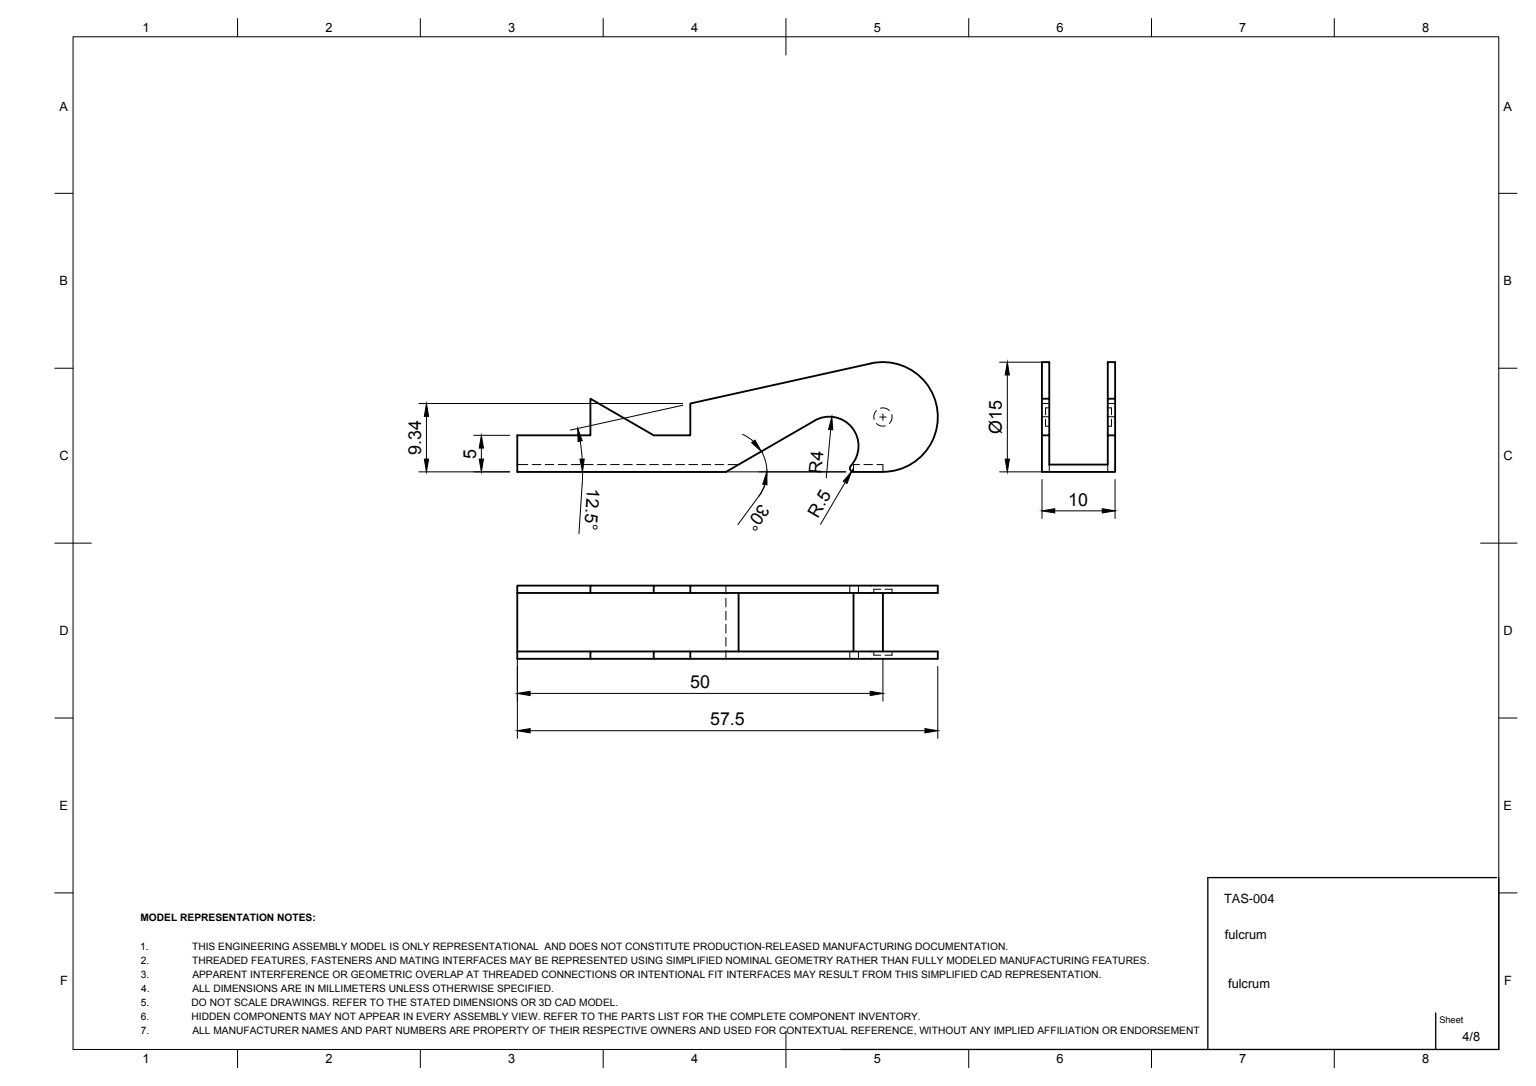
ISO-10303-21;
HEADER;
/* Generated by software containing ST-Developer
 * from STEP Tools, Inc. (www.steptools.com) 
 */

FILE_DESCRIPTION(
/* description */ ('STEP AP214'),
/* implementation_level */ '2;1');

FILE_NAME(
/* name */ 'fulcrum.step',
/* time_stamp */ '2026-11-04T19:48:07-08:00',
/* author */ (''),
/* organization */ (''),
/* preprocessor_version */ 'ST-DEVELOPER v20.2',
/* originating_system */ 'Autodesk Translation Framework v15.17.0.0',
/* authorisation */ '');

FILE_SCHEMA (('AUTOMOTIVE_DESIGN { 1 0 10303 214 3 1 1 }'));
ENDSEC;

DATA;
#10=MECHANICAL_DESIGN_GEOMETRIC_PRESENTATION_REPRESENTATION('',(#60),#9561);
#48=SHAPE_REPRESENTATION_RELATIONSHIP('SRR','None',#9588,#54);
#54=ADVANCED_BREP_SHAPE_REPRESENTATION('',(#66),#9556);
#60=STYLED_ITEM('',(#9627),#66);
#66=MANIFOLD_SOLID_BREP('Body1',#2406);
#77=FACE_BOUND('',#403,.T.);
#78=FACE_BOUND('',#405,.T.);
#100=PLANE('',#2558);
#101=PLANE('',#2559);
#102=PLANE('',#2560);
#103=PLANE('',#2561);
#104=PLANE('',#2562);
#105=PLANE('',#2563);
#106=PLANE('',#2564);
#107=PLANE('',#2568);
#108=PLANE('',#2569);
#109=PLANE('',#2570);
#110=PLANE('',#2571);
#111=PLANE('',#2572);
#112=PLANE('',#2573);
#113=PLANE('',#2574);
#114=PLANE('',#2575);
#115=PLANE('',#2576);
#116=PLANE('',#2578);
#117=PLANE('',#2579);
#118=PLANE('',#2582);
#119=PLANE('',#2583);
#120=PLANE('',#2584);
#121=PLANE('',#2585);
#122=PLANE('',#2586);
#123=PLANE('',#2587);
#124=PLANE('',#2588);
#125=PLANE('',#2589);
#223=FACE_OUTER_BOUND('',#372,.T.);
#224=FACE_OUTER_BOUND('',#373,.T.);
#225=FACE_OUTER_BOUND('',#374,.T.);
#226=FACE_OUTER_BOUND('',#375,.T.);
#227=FACE_OUTER_BOUND('',#376,.T.);
#228=FACE_OUTER_BOUND('',#377,.T.);
#229=FACE_OUTER_BOUND('',#378,.T.);
#230=FACE_OUTER_BOUND('',#379,.T.);
#231=FACE_OUTER_BOUND('',#380,.T.);
#232=FACE_OUTER_BOUND('',#381,.T.);
#233=FACE_OUTER_BOUND('',#382,.T.);
#234=FACE_OUTER_BOUND('',#383,.T.);
#235=FACE_OUTER_BOUND('',#384,.T.);
#236=FACE_OUTER_BOUND('',#385,.T.);
#237=FACE_OUTER_BOUND('',#386,.T.);
#238=FACE_OUTER_BOUND('',#387,.T.);
#239=FACE_OUTER_BOUND('',#388,.T.);
#240=FACE_OUTER_BOUND('',#389,.T.);
#241=FACE_OUTER_BOUND('',#390,.T.);
#242=FACE_OUTER_BOUND('',#391,.T.);
#243=FACE_OUTER_BOUND('',#392,.T.);
#244=FACE_OUTER_BOUND('',#393,.T.);
#245=FACE_OUTER_BOUND('',#394,.T.);
#246=FACE_OUTER_BOUND('',#395,.T.);
#247=FACE_OUTER_BOUND('',#396,.T.);
#248=FACE_OUTER_BOUND('',#397,.T.);
#249=FACE_OUTER_BOUND('',#398,.T.);
#250=FACE_OUTER_BOUND('',#399,.T.);
#251=FACE_OUTER_BOUND('',#400,.T.);
#252=FACE_OUTER_BOUND('',#401,.T.);
#253=FACE_OUTER_BOUND('',#402,.T.);
#254=FACE_OUTER_BOUND('',#404,.T.);
#255=FACE_OUTER_BOUND('',#406,.T.);
#256=FACE_OUTER_BOUND('',#407,.T.);
#372=EDGE_LOOP('',(#1733,#1734,#1735,#1736));
#373=EDGE_LOOP('',(#1737,#1738,#1739,#1740));
#374=EDGE_LOOP('',(#1741,#1742,#1743,#1744));
#375=EDGE_LOOP('',(#1745,#1746,#1747,#1748));
#376=EDGE_LOOP('',(#1749,#1750,#1751,#1752));
#377=EDGE_LOOP('',(#1753,#1754,#1755,#1756));
#378=EDGE_LOOP('',(#1757,#1758,#1759,#1760));
#379=EDGE_LOOP('',(#1761,#1762,#1763,#1764));
#380=EDGE_LOOP('',(#1765,#1766,#1767,#1768));
#381=EDGE_LOOP('',(#1769,#1770,#1771,#1772));
#382=EDGE_LOOP('',(#1773,#1774,#1775,#1776));
#383=EDGE_LOOP('',(#1777,#1778,#1779,#1780));
#384=EDGE_LOOP('',(#1781,#1782,#1783,#1784,#1785,#1786,#1787,#1788));
#385=EDGE_LOOP('',(#1789,#1790,#1791,#1792));
#386=EDGE_LOOP('',(#1793,#1794,#1795,#1796,#1797,#1798,#1799,#1800));
#387=EDGE_LOOP('',(#1801,#1802,#1803,#1804));
#388=EDGE_LOOP('',(#1805,#1806,#1807,#1808));
#389=EDGE_LOOP('',(#1809,#1810,#1811,#1812));
#390=EDGE_LOOP('',(#1813,#1814,#1815,#1816));
#391=EDGE_LOOP('',(#1817,#1818,#1819,#1820));
#392=EDGE_LOOP('',(#1821,#1822,#1823,#1824));
#393=EDGE_LOOP('',(#1825,#1826,#1827,#1828));
#394=EDGE_LOOP('',(#1829,#1830,#1831,#1832,#1833,#1834,#1835,#1836,#1837,
#1838,#1839,#1840,#1841));
#395=EDGE_LOOP('',(#1842,#1843,#1844,#1845,#1846,#1847,#1848,#1849,#1850,
#1851,#1852,#1853,#1854));
#396=EDGE_LOOP('',(#1855,#1856,#1857,#1858,#1859,#1860,#1861,#1862));
#397=EDGE_LOOP('',(#1863,#1864,#1865,#1866));
#398=EDGE_LOOP('',(#1867,#1868,#1869,#1870));
#399=EDGE_LOOP('',(#1871,#1872,#1873,#1874));
#400=EDGE_LOOP('',(#1875,#1876,#1877,#1878));
#401=EDGE_LOOP('',(#1879,#1880,#1881,#1882));
#402=EDGE_LOOP('',(#1883,#1884,#1885,#1886,#1887,#1888,#1889,#1890,#1891,
#1892,#1893,#1894,#1895,#1896,#1897));
#403=EDGE_LOOP('',(#1898));
#404=EDGE_LOOP('',(#1899,#1900,#1901,#1902,#1903,#1904,#1905,#1906,#1907,
#1908,#1909,#1910,#1911,#1912,#1913));
#405=EDGE_LOOP('',(#1914));
#406=EDGE_LOOP('',(#1915));
#407=EDGE_LOOP('',(#1916));
#540=LINE('',#3543,#790);
#541=LINE('',#3549,#791);
#542=LINE('',#3556,#792);
#543=LINE('',#3559,#793);
#544=LINE('',#3565,#794);
#545=LINE('',#3568,#795);
#546=LINE('',#3574,#796);
#547=LINE('',#3577,#797);
#548=LINE('',#3583,#798);
#549=LINE('',#3586,#799);
#550=LINE('',#3589,#800);
#551=LINE('',#3591,#801);
#552=LINE('',#3592,#802);
#553=LINE('',#3595,#803);
#554=LINE('',#3597,#804);
#555=LINE('',#3598,#805);
#556=LINE('',#3601,#806);
#557=LINE('',#3603,#807);
#558=LINE('',#3604,#808);
#559=LINE('',#3607,#809);
#560=LINE('',#3609,#810);
#561=LINE('',#3610,#811);
#562=LINE('',#3613,#812);
#563=LINE('',#3615,#813);
#564=LINE('',#3616,#814);
#565=LINE('',#3619,#815);
#566=LINE('',#3621,#816);
#567=LINE('',#3622,#817);
#568=LINE('',#3625,#818);
#569=LINE('',#3627,#819);
#570=LINE('',#3629,#820);
#571=LINE('',#3631,#821);
#572=LINE('',#3633,#822);
#573=LINE('',#3635,#823);
#574=LINE('',#3636,#824);
#575=LINE('',#3641,#825);
#576=LINE('',#3644,#826);
#577=LINE('',#3645,#827);
#578=LINE('',#3646,#828);
#579=LINE('',#3647,#829);
#580=LINE('',#3650,#830);
#581=LINE('',#3652,#831);
#582=LINE('',#3653,#832);
#583=LINE('',#3656,#833);
#584=LINE('',#3658,#834);
#585=LINE('',#3659,#835);
#586=LINE('',#3662,#836);
#587=LINE('',#3664,#837);
#588=LINE('',#3665,#838);
#589=LINE('',#3668,#839);
#590=LINE('',#3670,#840);
#591=LINE('',#3671,#841);
#592=LINE('',#3674,#842);
#593=LINE('',#3676,#843);
#594=LINE('',#3677,#844);
#595=LINE('',#3679,#845);
#596=LINE('',#3680,#846);
#597=LINE('',#3683,#847);
#598=LINE('',#3685,#848);
#599=LINE('',#3686,#849);
#600=LINE('',#3690,#850);
#601=LINE('',#3692,#851);
#602=LINE('',#3696,#852);
#603=LINE('',#3697,#853);
#604=LINE('',#3699,#854);
#605=LINE('',#3700,#855);
#606=LINE('',#3705,#856);
#607=LINE('',#3707,#857);
#608=LINE('',#3708,#858);
#609=LINE('',#3711,#859);
#610=LINE('',#3713,#860);
#611=LINE('',#3714,#861);
#612=LINE('',#3716,#862);
#613=LINE('',#3717,#863);
#614=LINE('',#3719,#864);
#615=LINE('',#3720,#865);
#790=VECTOR('',#2869,1.25);
#791=VECTOR('',#2876,1.25);
#792=VECTOR('',#2883,1000.);
#793=VECTOR('',#2886,1000.);
#794=VECTOR('',#2891,1000.);
#795=VECTOR('',#2894,1000.);
#796=VECTOR('',#2899,1000.);
#797=VECTOR('',#2902,1000.);
#798=VECTOR('',#2907,1000.);
#799=VECTOR('',#2910,1000.);
#800=VECTOR('',#2913,1000.);
#801=VECTOR('',#2914,1000.);
#802=VECTOR('',#2915,1000.);
#803=VECTOR('',#2918,1000.);
#804=VECTOR('',#2919,1000.);
#805=VECTOR('',#2920,1000.);
#806=VECTOR('',#2923,1000.);
#807=VECTOR('',#2924,1000.);
#808=VECTOR('',#2925,1000.);
#809=VECTOR('',#2928,1000.);
#810=VECTOR('',#2929,1000.);
#811=VECTOR('',#2930,1000.);
#812=VECTOR('',#2933,1000.);
#813=VECTOR('',#2934,1000.);
#814=VECTOR('',#2935,1000.);
#815=VECTOR('',#2938,1000.);
#816=VECTOR('',#2939,1000.);
#817=VECTOR('',#2940,1000.);
#818=VECTOR('',#2943,1000.);
#819=VECTOR('',#2944,1000.);
#820=VECTOR('',#2945,1000.);
#821=VECTOR('',#2946,1000.);
#822=VECTOR('',#2947,1000.);
#823=VECTOR('',#2948,1000.);
#824=VECTOR('',#2949,1000.);
#825=VECTOR('',#2954,1000.);
#826=VECTOR('',#2959,1000.);
#827=VECTOR('',#2960,1000.);
#828=VECTOR('',#2961,1000.);
#829=VECTOR('',#2962,1000.);
#830=VECTOR('',#2965,1000.);
#831=VECTOR('',#2966,1000.);
#832=VECTOR('',#2967,1000.);
#833=VECTOR('',#2970,1000.);
#834=VECTOR('',#2971,1000.);
#835=VECTOR('',#2972,1000.);
#836=VECTOR('',#2975,1000.);
#837=VECTOR('',#2976,1000.);
#838=VECTOR('',#2977,1000.);
#839=VECTOR('',#2980,1000.);
#840=VECTOR('',#2981,1000.);
#841=VECTOR('',#2982,1000.);
#842=VECTOR('',#2985,1000.);
#843=VECTOR('',#2986,1000.);
#844=VECTOR('',#2987,1000.);
#845=VECTOR('',#2990,1000.);
#846=VECTOR('',#2991,1000.);
#847=VECTOR('',#2994,1000.);
#848=VECTOR('',#2995,1000.);
#849=VECTOR('',#2996,1000.);
#850=VECTOR('',#3001,1000.);
#851=VECTOR('',#3004,1000.);
#852=VECTOR('',#3007,1000.);
#853=VECTOR('',#3008,1000.);
#854=VECTOR('',#3009,1000.);
#855=VECTOR('',#3010,1000.);
#856=VECTOR('',#3017,1000.);
#857=VECTOR('',#3018,1000.);
#858=VECTOR('',#3019,1000.);
#859=VECTOR('',#3022,1000.);
#860=VECTOR('',#3023,1000.);
#861=VECTOR('',#3024,1000.);
#862=VECTOR('',#3027,1000.);
#863=VECTOR('',#3028,1000.);
#864=VECTOR('',#3031,1000.);
#865=VECTOR('',#3032,1000.);
#1025=CIRCLE('',#2541,1.25);
#1026=CIRCLE('',#2542,1.25);
#1027=CIRCLE('',#2544,1.25);
#1028=CIRCLE('',#2545,1.25);
#1029=CIRCLE('',#2547,7.5);
#1030=CIRCLE('',#2548,7.5);
#1031=CIRCLE('',#2550,0.5);
#1032=CIRCLE('',#2551,0.5);
#1033=CIRCLE('',#2553,0.5);
#1034=CIRCLE('',#2554,0.5);
#1035=CIRCLE('',#2556,7.5);
#1036=CIRCLE('',#2557,7.5);
#1037=CIRCLE('',#2566,4.);
#1038=CIRCLE('',#2567,4.);
#1039=CIRCLE('',#2577,4.);
#1040=CIRCLE('',#2581,4.);
#1111=VERTEX_POINT('',#3540);
#1112=VERTEX_POINT('',#3542);
#1113=VERTEX_POINT('',#3546);
#1114=VERTEX_POINT('',#3548);
#1115=VERTEX_POINT('',#3552);
#1116=VERTEX_POINT('',#3553);
#1117=VERTEX_POINT('',#3555);
#1118=VERTEX_POINT('',#3557);
#1119=VERTEX_POINT('',#3561);
#1120=VERTEX_POINT('',#3562);
#1121=VERTEX_POINT('',#3564);
#1122=VERTEX_POINT('',#3566);
#1123=VERTEX_POINT('',#3570);
#1124=VERTEX_POINT('',#3571);
#1125=VERTEX_POINT('',#3573);
#1126=VERTEX_POINT('',#3575);
#1127=VERTEX_POINT('',#3579);
#1128=VERTEX_POINT('',#3580);
#1129=VERTEX_POINT('',#3582);
#1130=VERTEX_POINT('',#3584);
#1131=VERTEX_POINT('',#3588);
#1132=VERTEX_POINT('',#3590);
#1133=VERTEX_POINT('',#3594);
#1134=VERTEX_POINT('',#3596);
#1135=VERTEX_POINT('',#3600);
#1136=VERTEX_POINT('',#3602);
#1137=VERTEX_POINT('',#3606);
#1138=VERTEX_POINT('',#3608);
#1139=VERTEX_POINT('',#3612);
#1140=VERTEX_POINT('',#3614);
#1141=VERTEX_POINT('',#3618);
#1142=VERTEX_POINT('',#3620);
#1143=VERTEX_POINT('',#3624);
#1144=VERTEX_POINT('',#3626);
#1145=VERTEX_POINT('',#3628);
#1146=VERTEX_POINT('',#3630);
#1147=VERTEX_POINT('',#3632);
#1148=VERTEX_POINT('',#3634);
#1149=VERTEX_POINT('',#3638);
#1150=VERTEX_POINT('',#3640);
#1151=VERTEX_POINT('',#3649);
#1152=VERTEX_POINT('',#3651);
#1153=VERTEX_POINT('',#3655);
#1154=VERTEX_POINT('',#3657);
#1155=VERTEX_POINT('',#3661);
#1156=VERTEX_POINT('',#3663);
#1157=VERTEX_POINT('',#3667);
#1158=VERTEX_POINT('',#3669);
#1159=VERTEX_POINT('',#3673);
#1160=VERTEX_POINT('',#3675);
#1161=VERTEX_POINT('',#3682);
#1162=VERTEX_POINT('',#3684);
#1163=VERTEX_POINT('',#3688);
#1164=VERTEX_POINT('',#3694);
#1165=VERTEX_POINT('',#3695);
#1166=VERTEX_POINT('',#3698);
#1167=VERTEX_POINT('',#3704);
#1168=VERTEX_POINT('',#3706);
#1169=VERTEX_POINT('',#3710);
#1170=VERTEX_POINT('',#3712);
#1334=EDGE_CURVE('',#1111,#1111,#1025,.T.);
#1335=EDGE_CURVE('',#1111,#1112,#540,.T.);
#1336=EDGE_CURVE('',#1112,#1112,#1026,.T.);
#1337=EDGE_CURVE('',#1113,#1113,#1027,.T.);
#1338=EDGE_CURVE('',#1113,#1114,#541,.T.);
#1339=EDGE_CURVE('',#1114,#1114,#1028,.T.);
#1340=EDGE_CURVE('',#1115,#1116,#1029,.T.);
#1341=EDGE_CURVE('',#1115,#1117,#542,.T.);
#1342=EDGE_CURVE('',#1117,#1118,#1030,.T.);
#1343=EDGE_CURVE('',#1116,#1118,#543,.T.);
#1344=EDGE_CURVE('',#1119,#1120,#1031,.T.);
#1345=EDGE_CURVE('',#1121,#1120,#544,.T.);
#1346=EDGE_CURVE('',#1122,#1121,#1032,.T.);
#1347=EDGE_CURVE('',#1119,#1122,#545,.T.);
#1348=EDGE_CURVE('',#1123,#1124,#1033,.T.);
#1349=EDGE_CURVE('',#1125,#1123,#546,.T.);
#1350=EDGE_CURVE('',#1125,#1126,#1034,.T.);
#1351=EDGE_CURVE('',#1124,#1126,#547,.T.);
#1352=EDGE_CURVE('',#1127,#1128,#1035,.T.);
#1353=EDGE_CURVE('',#1127,#1129,#548,.T.);
#1354=EDGE_CURVE('',#1129,#1130,#1036,.T.);
#1355=EDGE_CURVE('',#1128,#1130,#549,.T.);
#1356=EDGE_CURVE('',#1128,#1131,#550,.T.);
#1357=EDGE_CURVE('',#1130,#1132,#551,.T.);
#1358=EDGE_CURVE('',#1131,#1132,#552,.T.);
#1359=EDGE_CURVE('',#1131,#1133,#553,.T.);
#1360=EDGE_CURVE('',#1132,#1134,#554,.T.);
#1361=EDGE_CURVE('',#1133,#1134,#555,.T.);
#1362=EDGE_CURVE('',#1133,#1135,#556,.T.);
#1363=EDGE_CURVE('',#1134,#1136,#557,.T.);
#1364=EDGE_CURVE('',#1135,#1136,#558,.T.);
#1365=EDGE_CURVE('',#1135,#1137,#559,.T.);
#1366=EDGE_CURVE('',#1136,#1138,#560,.T.);
#1367=EDGE_CURVE('',#1137,#1138,#561,.T.);
#1368=EDGE_CURVE('',#1137,#1139,#562,.T.);
#1369=EDGE_CURVE('',#1138,#1140,#563,.T.);
#1370=EDGE_CURVE('',#1139,#1140,#564,.T.);
#1371=EDGE_CURVE('',#1139,#1141,#565,.T.);
#1372=EDGE_CURVE('',#1140,#1142,#566,.T.);
#1373=EDGE_CURVE('',#1141,#1142,#567,.T.);
#1374=EDGE_CURVE('',#1141,#1143,#568,.T.);
#1375=EDGE_CURVE('',#1142,#1144,#569,.T.);
#1376=EDGE_CURVE('',#1145,#1144,#570,.T.);
#1377=EDGE_CURVE('',#1146,#1145,#571,.T.);
#1378=EDGE_CURVE('',#1146,#1147,#572,.T.);
#1379=EDGE_CURVE('',#1147,#1148,#573,.T.);
#1380=EDGE_CURVE('',#1148,#1143,#574,.T.);
#1381=EDGE_CURVE('',#1126,#1149,#1037,.T.);
#1382=EDGE_CURVE('',#1150,#1149,#575,.T.);
#1383=EDGE_CURVE('',#1124,#1150,#1038,.T.);
#1384=EDGE_CURVE('',#1121,#1115,#576,.T.);
#1385=EDGE_CURVE('',#1120,#1125,#577,.T.);
#1386=EDGE_CURVE('',#1123,#1129,#578,.T.);
#1387=EDGE_CURVE('',#1117,#1127,#579,.T.);
#1388=EDGE_CURVE('',#1118,#1151,#580,.T.);
#1389=EDGE_CURVE('',#1152,#1151,#581,.T.);
#1390=EDGE_CURVE('',#1116,#1152,#582,.T.);
#1391=EDGE_CURVE('',#1151,#1153,#583,.T.);
#1392=EDGE_CURVE('',#1154,#1153,#584,.T.);
#1393=EDGE_CURVE('',#1152,#1154,#585,.T.);
#1394=EDGE_CURVE('',#1153,#1155,#586,.T.);
#1395=EDGE_CURVE('',#1156,#1155,#587,.T.);
#1396=EDGE_CURVE('',#1154,#1156,#588,.T.);
#1397=EDGE_CURVE('',#1155,#1157,#589,.T.);
#1398=EDGE_CURVE('',#1158,#1157,#590,.T.);
#1399=EDGE_CURVE('',#1156,#1158,#591,.T.);
#1400=EDGE_CURVE('',#1157,#1159,#592,.T.);
#1401=EDGE_CURVE('',#1160,#1159,#593,.T.);
#1402=EDGE_CURVE('',#1158,#1160,#594,.T.);
#1403=EDGE_CURVE('',#1159,#1147,#595,.T.);
#1404=EDGE_CURVE('',#1160,#1146,#596,.T.);
#1405=EDGE_CURVE('',#1144,#1161,#597,.T.);
#1406=EDGE_CURVE('',#1161,#1162,#598,.T.);
#1407=EDGE_CURVE('',#1145,#1162,#599,.T.);
#1408=EDGE_CURVE('',#1122,#1163,#1039,.T.);
#1409=EDGE_CURVE('',#1163,#1162,#600,.T.);
#1410=EDGE_CURVE('',#1150,#1161,#601,.T.);
#1411=EDGE_CURVE('',#1164,#1165,#602,.T.);
#1412=EDGE_CURVE('',#1164,#1163,#603,.T.);
#1413=EDGE_CURVE('',#1149,#1166,#604,.T.);
#1414=EDGE_CURVE('',#1166,#1165,#605,.T.);
#1415=EDGE_CURVE('',#1119,#1164,#1040,.T.);
#1416=EDGE_CURVE('',#1167,#1120,#606,.T.);
#1417=EDGE_CURVE('',#1167,#1168,#607,.T.);
#1418=EDGE_CURVE('',#1168,#1125,#608,.T.);
#1419=EDGE_CURVE('',#1169,#1127,#609,.T.);
#1420=EDGE_CURVE('',#1170,#1169,#610,.T.);
#1421=EDGE_CURVE('',#1170,#1117,#611,.T.);
#1422=EDGE_CURVE('',#1167,#1170,#612,.T.);
#1423=EDGE_CURVE('',#1168,#1169,#613,.T.);
#1424=EDGE_CURVE('',#1143,#1166,#614,.T.);
#1425=EDGE_CURVE('',#1148,#1165,#615,.T.);
#1733=ORIENTED_EDGE('',*,*,#1334,.T.);
#1734=ORIENTED_EDGE('',*,*,#1335,.T.);
#1735=ORIENTED_EDGE('',*,*,#1336,.T.);
#1736=ORIENTED_EDGE('',*,*,#1335,.F.);
#1737=ORIENTED_EDGE('',*,*,#1337,.F.);
#1738=ORIENTED_EDGE('',*,*,#1338,.T.);
#1739=ORIENTED_EDGE('',*,*,#1339,.F.);
#1740=ORIENTED_EDGE('',*,*,#1338,.F.);
#1741=ORIENTED_EDGE('',*,*,#1340,.F.);
#1742=ORIENTED_EDGE('',*,*,#1341,.T.);
#1743=ORIENTED_EDGE('',*,*,#1342,.T.);
#1744=ORIENTED_EDGE('',*,*,#1343,.F.);
#1745=ORIENTED_EDGE('',*,*,#1344,.T.);
#1746=ORIENTED_EDGE('',*,*,#1345,.F.);
#1747=ORIENTED_EDGE('',*,*,#1346,.F.);
#1748=ORIENTED_EDGE('',*,*,#1347,.F.);
#1749=ORIENTED_EDGE('',*,*,#1348,.F.);
#1750=ORIENTED_EDGE('',*,*,#1349,.F.);
#1751=ORIENTED_EDGE('',*,*,#1350,.T.);
#1752=ORIENTED_EDGE('',*,*,#1351,.F.);
#1753=ORIENTED_EDGE('',*,*,#1352,.F.);
#1754=ORIENTED_EDGE('',*,*,#1353,.T.);
#1755=ORIENTED_EDGE('',*,*,#1354,.T.);
#1756=ORIENTED_EDGE('',*,*,#1355,.F.);
#1757=ORIENTED_EDGE('',*,*,#1356,.F.);
#1758=ORIENTED_EDGE('',*,*,#1355,.T.);
#1759=ORIENTED_EDGE('',*,*,#1357,.T.);
#1760=ORIENTED_EDGE('',*,*,#1358,.F.);
#1761=ORIENTED_EDGE('',*,*,#1359,.F.);
#1762=ORIENTED_EDGE('',*,*,#1358,.T.);
#1763=ORIENTED_EDGE('',*,*,#1360,.T.);
#1764=ORIENTED_EDGE('',*,*,#1361,.F.);
#1765=ORIENTED_EDGE('',*,*,#1362,.F.);
#1766=ORIENTED_EDGE('',*,*,#1361,.T.);
#1767=ORIENTED_EDGE('',*,*,#1363,.T.);
#1768=ORIENTED_EDGE('',*,*,#1364,.F.);
#1769=ORIENTED_EDGE('',*,*,#1365,.F.);
#1770=ORIENTED_EDGE('',*,*,#1364,.T.);
#1771=ORIENTED_EDGE('',*,*,#1366,.T.);
#1772=ORIENTED_EDGE('',*,*,#1367,.F.);
#1773=ORIENTED_EDGE('',*,*,#1368,.F.);
#1774=ORIENTED_EDGE('',*,*,#1367,.T.);
#1775=ORIENTED_EDGE('',*,*,#1369,.T.);
#1776=ORIENTED_EDGE('',*,*,#1370,.F.);
#1777=ORIENTED_EDGE('',*,*,#1371,.F.);
#1778=ORIENTED_EDGE('',*,*,#1370,.T.);
#1779=ORIENTED_EDGE('',*,*,#1372,.T.);
#1780=ORIENTED_EDGE('',*,*,#1373,.F.);
#1781=ORIENTED_EDGE('',*,*,#1374,.F.);
#1782=ORIENTED_EDGE('',*,*,#1373,.T.);
#1783=ORIENTED_EDGE('',*,*,#1375,.T.);
#1784=ORIENTED_EDGE('',*,*,#1376,.F.);
#1785=ORIENTED_EDGE('',*,*,#1377,.F.);
#1786=ORIENTED_EDGE('',*,*,#1378,.T.);
#1787=ORIENTED_EDGE('',*,*,#1379,.T.);
#1788=ORIENTED_EDGE('',*,*,#1380,.T.);
#1789=ORIENTED_EDGE('',*,*,#1351,.T.);
#1790=ORIENTED_EDGE('',*,*,#1381,.T.);
#1791=ORIENTED_EDGE('',*,*,#1382,.F.);
#1792=ORIENTED_EDGE('',*,*,#1383,.F.);
#1793=ORIENTED_EDGE('',*,*,#1384,.F.);
#1794=ORIENTED_EDGE('',*,*,#1345,.T.);
#1795=ORIENTED_EDGE('',*,*,#1385,.T.);
#1796=ORIENTED_EDGE('',*,*,#1349,.T.);
#1797=ORIENTED_EDGE('',*,*,#1386,.T.);
#1798=ORIENTED_EDGE('',*,*,#1353,.F.);
#1799=ORIENTED_EDGE('',*,*,#1387,.F.);
#1800=ORIENTED_EDGE('',*,*,#1341,.F.);
#1801=ORIENTED_EDGE('',*,*,#1343,.T.);
#1802=ORIENTED_EDGE('',*,*,#1388,.T.);
#1803=ORIENTED_EDGE('',*,*,#1389,.F.);
#1804=ORIENTED_EDGE('',*,*,#1390,.F.);
#1805=ORIENTED_EDGE('',*,*,#1389,.T.);
#1806=ORIENTED_EDGE('',*,*,#1391,.T.);
#1807=ORIENTED_EDGE('',*,*,#1392,.F.);
#1808=ORIENTED_EDGE('',*,*,#1393,.F.);
#1809=ORIENTED_EDGE('',*,*,#1392,.T.);
#1810=ORIENTED_EDGE('',*,*,#1394,.T.);
#1811=ORIENTED_EDGE('',*,*,#1395,.F.);
#1812=ORIENTED_EDGE('',*,*,#1396,.F.);
#1813=ORIENTED_EDGE('',*,*,#1395,.T.);
#1814=ORIENTED_EDGE('',*,*,#1397,.T.);
#1815=ORIENTED_EDGE('',*,*,#1398,.F.);
#1816=ORIENTED_EDGE('',*,*,#1399,.F.);
#1817=ORIENTED_EDGE('',*,*,#1398,.T.);
#1818=ORIENTED_EDGE('',*,*,#1400,.T.);
#1819=ORIENTED_EDGE('',*,*,#1401,.F.);
#1820=ORIENTED_EDGE('',*,*,#1402,.F.);
#1821=ORIENTED_EDGE('',*,*,#1401,.T.);
#1822=ORIENTED_EDGE('',*,*,#1403,.T.);
#1823=ORIENTED_EDGE('',*,*,#1378,.F.);
#1824=ORIENTED_EDGE('',*,*,#1404,.F.);
#1825=ORIENTED_EDGE('',*,*,#1405,.T.);
#1826=ORIENTED_EDGE('',*,*,#1406,.T.);
#1827=ORIENTED_EDGE('',*,*,#1407,.F.);
#1828=ORIENTED_EDGE('',*,*,#1376,.T.);
#1829=ORIENTED_EDGE('',*,*,#1408,.F.);
#1830=ORIENTED_EDGE('',*,*,#1346,.T.);
#1831=ORIENTED_EDGE('',*,*,#1384,.T.);
#1832=ORIENTED_EDGE('',*,*,#1340,.T.);
#1833=ORIENTED_EDGE('',*,*,#1390,.T.);
#1834=ORIENTED_EDGE('',*,*,#1393,.T.);
#1835=ORIENTED_EDGE('',*,*,#1396,.T.);
#1836=ORIENTED_EDGE('',*,*,#1399,.T.);
#1837=ORIENTED_EDGE('',*,*,#1402,.T.);
#1838=ORIENTED_EDGE('',*,*,#1404,.T.);
#1839=ORIENTED_EDGE('',*,*,#1377,.T.);
#1840=ORIENTED_EDGE('',*,*,#1407,.T.);
#1841=ORIENTED_EDGE('',*,*,#1409,.F.);
#1842=ORIENTED_EDGE('',*,*,#1386,.F.);
#1843=ORIENTED_EDGE('',*,*,#1348,.T.);
#1844=ORIENTED_EDGE('',*,*,#1383,.T.);
#1845=ORIENTED_EDGE('',*,*,#1410,.T.);
#1846=ORIENTED_EDGE('',*,*,#1405,.F.);
#1847=ORIENTED_EDGE('',*,*,#1375,.F.);
#1848=ORIENTED_EDGE('',*,*,#1372,.F.);
#1849=ORIENTED_EDGE('',*,*,#1369,.F.);
#1850=ORIENTED_EDGE('',*,*,#1366,.F.);
#1851=ORIENTED_EDGE('',*,*,#1363,.F.);
#1852=ORIENTED_EDGE('',*,*,#1360,.F.);
#1853=ORIENTED_EDGE('',*,*,#1357,.F.);
#1854=ORIENTED_EDGE('',*,*,#1354,.F.);
#1855=ORIENTED_EDGE('',*,*,#1411,.F.);
#1856=ORIENTED_EDGE('',*,*,#1412,.T.);
#1857=ORIENTED_EDGE('',*,*,#1409,.T.);
#1858=ORIENTED_EDGE('',*,*,#1406,.F.);
#1859=ORIENTED_EDGE('',*,*,#1410,.F.);
#1860=ORIENTED_EDGE('',*,*,#1382,.T.);
#1861=ORIENTED_EDGE('',*,*,#1413,.T.);
#1862=ORIENTED_EDGE('',*,*,#1414,.T.);
#1863=ORIENTED_EDGE('',*,*,#1415,.F.);
#1864=ORIENTED_EDGE('',*,*,#1347,.T.);
#1865=ORIENTED_EDGE('',*,*,#1408,.T.);
#1866=ORIENTED_EDGE('',*,*,#1412,.F.);
#1867=ORIENTED_EDGE('',*,*,#1385,.F.);
#1868=ORIENTED_EDGE('',*,*,#1416,.F.);
#1869=ORIENTED_EDGE('',*,*,#1417,.T.);
#1870=ORIENTED_EDGE('',*,*,#1418,.T.);
#1871=ORIENTED_EDGE('',*,*,#1387,.T.);
#1872=ORIENTED_EDGE('',*,*,#1419,.F.);
#1873=ORIENTED_EDGE('',*,*,#1420,.F.);
#1874=ORIENTED_EDGE('',*,*,#1421,.T.);
#1875=ORIENTED_EDGE('',*,*,#1422,.T.);
#1876=ORIENTED_EDGE('',*,*,#1420,.T.);
#1877=ORIENTED_EDGE('',*,*,#1423,.F.);
#1878=ORIENTED_EDGE('',*,*,#1417,.F.);
#1879=ORIENTED_EDGE('',*,*,#1424,.F.);
#1880=ORIENTED_EDGE('',*,*,#1380,.F.);
#1881=ORIENTED_EDGE('',*,*,#1425,.T.);
#1882=ORIENTED_EDGE('',*,*,#1414,.F.);
#1883=ORIENTED_EDGE('',*,*,#1415,.T.);
#1884=ORIENTED_EDGE('',*,*,#1411,.T.);
#1885=ORIENTED_EDGE('',*,*,#1425,.F.);
#1886=ORIENTED_EDGE('',*,*,#1379,.F.);
#1887=ORIENTED_EDGE('',*,*,#1403,.F.);
#1888=ORIENTED_EDGE('',*,*,#1400,.F.);
#1889=ORIENTED_EDGE('',*,*,#1397,.F.);
#1890=ORIENTED_EDGE('',*,*,#1394,.F.);
#1891=ORIENTED_EDGE('',*,*,#1391,.F.);
#1892=ORIENTED_EDGE('',*,*,#1388,.F.);
#1893=ORIENTED_EDGE('',*,*,#1342,.F.);
#1894=ORIENTED_EDGE('',*,*,#1421,.F.);
#1895=ORIENTED_EDGE('',*,*,#1422,.F.);
#1896=ORIENTED_EDGE('',*,*,#1416,.T.);
#1897=ORIENTED_EDGE('',*,*,#1344,.F.);
#1898=ORIENTED_EDGE('',*,*,#1334,.F.);
#1899=ORIENTED_EDGE('',*,*,#1423,.T.);
#1900=ORIENTED_EDGE('',*,*,#1419,.T.);
#1901=ORIENTED_EDGE('',*,*,#1352,.T.);
#1902=ORIENTED_EDGE('',*,*,#1356,.T.);
#1903=ORIENTED_EDGE('',*,*,#1359,.T.);
#1904=ORIENTED_EDGE('',*,*,#1362,.T.);
#1905=ORIENTED_EDGE('',*,*,#1365,.T.);
#1906=ORIENTED_EDGE('',*,*,#1368,.T.);
#1907=ORIENTED_EDGE('',*,*,#1371,.T.);
#1908=ORIENTED_EDGE('',*,*,#1374,.T.);
#1909=ORIENTED_EDGE('',*,*,#1424,.T.);
#1910=ORIENTED_EDGE('',*,*,#1413,.F.);
#1911=ORIENTED_EDGE('',*,*,#1381,.F.);
#1912=ORIENTED_EDGE('',*,*,#1350,.F.);
#1913=ORIENTED_EDGE('',*,*,#1418,.F.);
#1914=ORIENTED_EDGE('',*,*,#1339,.T.);
#1915=ORIENTED_EDGE('',*,*,#1337,.T.);
#1916=ORIENTED_EDGE('',*,*,#1336,.F.);
#2246=CYLINDRICAL_SURFACE('',#2540,1.25);
#2247=CYLINDRICAL_SURFACE('',#2543,1.25);
#2248=CYLINDRICAL_SURFACE('',#2546,7.5);
#2249=CYLINDRICAL_SURFACE('',#2549,0.5);
#2250=CYLINDRICAL_SURFACE('',#2552,0.5);
#2251=CYLINDRICAL_SURFACE('',#2555,7.5);
#2252=CYLINDRICAL_SURFACE('',#2565,4.);
#2253=CYLINDRICAL_SURFACE('',#2580,4.);
#2291=ADVANCED_FACE('',(#223),#2246,.F.);
#2292=ADVANCED_FACE('',(#224),#2247,.F.);
#2293=ADVANCED_FACE('',(#225),#2248,.T.);
#2294=ADVANCED_FACE('',(#226),#2249,.T.);
#2295=ADVANCED_FACE('',(#227),#2250,.T.);
#2296=ADVANCED_FACE('',(#228),#2251,.T.);
#2297=ADVANCED_FACE('',(#229),#100,.F.);
#2298=ADVANCED_FACE('',(#230),#101,.F.);
#2299=ADVANCED_FACE('',(#231),#102,.F.);
#2300=ADVANCED_FACE('',(#232),#103,.F.);
#2301=ADVANCED_FACE('',(#233),#104,.F.);
#2302=ADVANCED_FACE('',(#234),#105,.F.);
#2303=ADVANCED_FACE('',(#235),#106,.F.);
#2304=ADVANCED_FACE('',(#236),#2252,.F.);
#2305=ADVANCED_FACE('',(#237),#107,.F.);
#2306=ADVANCED_FACE('',(#238),#108,.F.);
#2307=ADVANCED_FACE('',(#239),#109,.F.);
#2308=ADVANCED_FACE('',(#240),#110,.F.);
#2309=ADVANCED_FACE('',(#241),#111,.F.);
#2310=ADVANCED_FACE('',(#242),#112,.F.);
#2311=ADVANCED_FACE('',(#243),#113,.F.);
#2312=ADVANCED_FACE('',(#244),#114,.F.);
#2313=ADVANCED_FACE('',(#245),#115,.F.);
#2314=ADVANCED_FACE('',(#246),#116,.T.);
#2315=ADVANCED_FACE('',(#247),#117,.T.);
#2316=ADVANCED_FACE('',(#248),#2253,.F.);
#2317=ADVANCED_FACE('',(#249),#118,.T.);
#2318=ADVANCED_FACE('',(#250),#119,.F.);
#2319=ADVANCED_FACE('',(#251),#120,.T.);
#2320=ADVANCED_FACE('',(#252),#121,.T.);
#2321=ADVANCED_FACE('',(#253,#77),#122,.T.);
#2322=ADVANCED_FACE('',(#254,#78),#123,.F.);
#2323=ADVANCED_FACE('',(#255),#124,.T.);
#2324=ADVANCED_FACE('',(#256),#125,.F.);
#2406=CLOSED_SHELL('',(#2291,#2292,#2293,#2294,#2295,#2296,#2297,#2298,
#2299,#2300,#2301,#2302,#2303,#2304,#2305,#2306,#2307,#2308,#2309,#2310,
#2311,#2312,#2313,#2314,#2315,#2316,#2317,#2318,#2319,#2320,#2321,#2322,
#2323,#2324));
#2539=AXIS2_PLACEMENT_3D('',#3538,#2863,#2864);
#2540=AXIS2_PLACEMENT_3D('',#3539,#2865,#2866);
#2541=AXIS2_PLACEMENT_3D('',#3541,#2867,#2868);
#2542=AXIS2_PLACEMENT_3D('',#3544,#2870,#2871);
#2543=AXIS2_PLACEMENT_3D('',#3545,#2872,#2873);
#2544=AXIS2_PLACEMENT_3D('',#3547,#2874,#2875);
#2545=AXIS2_PLACEMENT_3D('',#3550,#2877,#2878);
#2546=AXIS2_PLACEMENT_3D('',#3551,#2879,#2880);
#2547=AXIS2_PLACEMENT_3D('',#3554,#2881,#2882);
#2548=AXIS2_PLACEMENT_3D('',#3558,#2884,#2885);
#2549=AXIS2_PLACEMENT_3D('',#3560,#2887,#2888);
#2550=AXIS2_PLACEMENT_3D('',#3563,#2889,#2890);
#2551=AXIS2_PLACEMENT_3D('',#3567,#2892,#2893);
#2552=AXIS2_PLACEMENT_3D('',#3569,#2895,#2896);
#2553=AXIS2_PLACEMENT_3D('',#3572,#2897,#2898);
#2554=AXIS2_PLACEMENT_3D('',#3576,#2900,#2901);
#2555=AXIS2_PLACEMENT_3D('',#3578,#2903,#2904);
#2556=AXIS2_PLACEMENT_3D('',#3581,#2905,#2906);
#2557=AXIS2_PLACEMENT_3D('',#3585,#2908,#2909);
#2558=AXIS2_PLACEMENT_3D('',#3587,#2911,#2912);
#2559=AXIS2_PLACEMENT_3D('',#3593,#2916,#2917);
#2560=AXIS2_PLACEMENT_3D('',#3599,#2921,#2922);
#2561=AXIS2_PLACEMENT_3D('',#3605,#2926,#2927);
#2562=AXIS2_PLACEMENT_3D('',#3611,#2931,#2932);
#2563=AXIS2_PLACEMENT_3D('',#3617,#2936,#2937);
#2564=AXIS2_PLACEMENT_3D('',#3623,#2941,#2942);
#2565=AXIS2_PLACEMENT_3D('',#3637,#2950,#2951);
#2566=AXIS2_PLACEMENT_3D('',#3639,#2952,#2953);
#2567=AXIS2_PLACEMENT_3D('',#3642,#2955,#2956);
#2568=AXIS2_PLACEMENT_3D('',#3643,#2957,#2958);
#2569=AXIS2_PLACEMENT_3D('',#3648,#2963,#2964);
#2570=AXIS2_PLACEMENT_3D('',#3654,#2968,#2969);
#2571=AXIS2_PLACEMENT_3D('',#3660,#2973,#2974);
#2572=AXIS2_PLACEMENT_3D('',#3666,#2978,#2979);
#2573=AXIS2_PLACEMENT_3D('',#3672,#2983,#2984);
#2574=AXIS2_PLACEMENT_3D('',#3678,#2988,#2989);
#2575=AXIS2_PLACEMENT_3D('',#3681,#2992,#2993);
#2576=AXIS2_PLACEMENT_3D('',#3687,#2997,#2998);
#2577=AXIS2_PLACEMENT_3D('',#3689,#2999,#3000);
#2578=AXIS2_PLACEMENT_3D('',#3691,#3002,#3003);
#2579=AXIS2_PLACEMENT_3D('',#3693,#3005,#3006);
#2580=AXIS2_PLACEMENT_3D('',#3701,#3011,#3012);
#2581=AXIS2_PLACEMENT_3D('',#3702,#3013,#3014);
#2582=AXIS2_PLACEMENT_3D('',#3703,#3015,#3016);
#2583=AXIS2_PLACEMENT_3D('',#3709,#3020,#3021);
#2584=AXIS2_PLACEMENT_3D('',#3715,#3025,#3026);
#2585=AXIS2_PLACEMENT_3D('',#3718,#3029,#3030);
#2586=AXIS2_PLACEMENT_3D('',#3721,#3033,#3034);
#2587=AXIS2_PLACEMENT_3D('',#3722,#3035,#3036);
#2588=AXIS2_PLACEMENT_3D('',#3723,#3037,#3038);
#2589=AXIS2_PLACEMENT_3D('',#3724,#3039,#3040);
#2863=DIRECTION('axis',(0.,0.,1.));
#2864=DIRECTION('refdir',(1.,0.,0.));
#2865=DIRECTION('center_axis',(0.,0.,1.));
#2866=DIRECTION('ref_axis',(1.,0.,0.));
#2867=DIRECTION('center_axis',(0.,0.,-1.));
#2868=DIRECTION('ref_axis',(-1.,0.,0.));
#2869=DIRECTION('',(0.,0.,1.));
#2870=DIRECTION('center_axis',(0.,0.,1.));
#2871=DIRECTION('ref_axis',(1.,0.,0.));
#2872=DIRECTION('center_axis',(0.,0.,1.));
#2873=DIRECTION('ref_axis',(1.,0.,0.));
#2874=DIRECTION('center_axis',(0.,0.,1.));
#2875=DIRECTION('ref_axis',(1.,0.,0.));
#2876=DIRECTION('',(0.,0.,1.));
#2877=DIRECTION('center_axis',(0.,0.,-1.));
#2878=DIRECTION('ref_axis',(-1.,0.,0.));
#2879=DIRECTION('center_axis',(0.,0.,-1.));
#2880=DIRECTION('ref_axis',(-1.,0.,0.));
#2881=DIRECTION('center_axis',(0.,0.,1.));
#2882=DIRECTION('ref_axis',(-1.,0.,0.));
#2883=DIRECTION('',(0.,0.,-1.));
#2884=DIRECTION('center_axis',(0.,0.,1.));
#2885=DIRECTION('ref_axis',(-1.,0.,0.));
#2886=DIRECTION('',(0.,0.,-1.));
#2887=DIRECTION('center_axis',(0.,0.,1.));
#2888=DIRECTION('ref_axis',(1.,0.,0.));
#2889=DIRECTION('center_axis',(0.,0.,1.));
#2890=DIRECTION('ref_axis',(-1.,8.67361737988404E-16,0.));
#2891=DIRECTION('',(0.,0.,-1.));
#2892=DIRECTION('center_axis',(0.,0.,1.));
#2893=DIRECTION('ref_axis',(-1.,8.67361737988404E-16,0.));
#2894=DIRECTION('',(0.,0.,1.));
#2895=DIRECTION('center_axis',(0.,0.,1.));
#2896=DIRECTION('ref_axis',(1.,0.,0.));
#2897=DIRECTION('center_axis',(0.,0.,-1.));
#2898=DIRECTION('ref_axis',(-1.,0.,0.));
#2899=DIRECTION('',(0.,0.,-1.));
#2900=DIRECTION('center_axis',(0.,0.,-1.));
#2901=DIRECTION('ref_axis',(-1.,0.,0.));
#2902=DIRECTION('',(0.,0.,1.));
#2903=DIRECTION('center_axis',(0.,0.,-1.));
#2904=DIRECTION('ref_axis',(-1.,0.,0.));
#2905=DIRECTION('center_axis',(0.,0.,1.));
#2906=DIRECTION('ref_axis',(-1.,0.,0.));
#2907=DIRECTION('',(0.,0.,-1.));
#2908=DIRECTION('center_axis',(0.,0.,1.));
#2909=DIRECTION('ref_axis',(-1.,0.,0.));
#2910=DIRECTION('',(0.,0.,-1.));
#2911=DIRECTION('center_axis',(0.537299608346827,0.843391445812884,0.));
#2912=DIRECTION('ref_axis',(-0.843391445812884,0.537299608346827,0.));
#2913=DIRECTION('',(0.843391445812883,-0.537299608346827,0.));
#2914=DIRECTION('',(0.843391445812883,-0.537299608346827,0.));
#2915=DIRECTION('',(0.,0.,-1.));
#2916=DIRECTION('center_axis',(-0.707106781186552,0.707106781186543,0.));
#2917=DIRECTION('ref_axis',(-0.707106781186543,-0.707106781186552,0.));
#2918=DIRECTION('',(0.707106781186543,0.707106781186552,0.));
#2919=DIRECTION('',(0.707106781186543,0.707106781186552,0.));
#2920=DIRECTION('',(0.,0.,-1.));
#2921=DIRECTION('center_axis',(0.707106781186547,0.707106781186548,0.));
#2922=DIRECTION('ref_axis',(-0.707106781186548,0.707106781186547,0.));
#2923=DIRECTION('',(0.707106781186548,-0.707106781186547,0.));
#2924=DIRECTION('',(0.707106781186548,-0.707106781186547,0.));
#2925=DIRECTION('',(0.,0.,-1.));
#2926=DIRECTION('center_axis',(0.965925826289068,0.258819045102523,0.));
#2927=DIRECTION('ref_axis',(-0.258819045102523,0.965925826289068,0.));
#2928=DIRECTION('',(0.258819045102523,-0.965925826289068,0.));
#2929=DIRECTION('',(0.258819045102523,-0.965925826289068,0.));
#2930=DIRECTION('',(0.,0.,-1.));
#2931=DIRECTION('center_axis',(-0.707106781186541,0.707106781186554,0.));
#2932=DIRECTION('ref_axis',(-0.707106781186554,-0.707106781186541,0.));
#2933=DIRECTION('',(0.707106781186554,0.707106781186541,0.));
#2934=DIRECTION('',(0.707106781186554,0.707106781186541,0.));
#2935=DIRECTION('',(0.,0.,-1.));
#2936=DIRECTION('center_axis',(0.707106781186545,0.70710678118655,0.));
#2937=DIRECTION('ref_axis',(-0.70710678118655,0.707106781186545,0.));
#2938=DIRECTION('',(0.70710678118655,-0.707106781186545,0.));
#2939=DIRECTION('',(0.70710678118655,-0.707106781186545,0.));
#2940=DIRECTION('',(0.,0.,-1.));
#2941=DIRECTION('center_axis',(-0.707106781186549,0.707106781186546,0.));
#2942=DIRECTION('ref_axis',(-0.707106781186546,-0.707106781186549,0.));
#2943=DIRECTION('',(0.707106781186546,0.707106781186549,0.));
#2944=DIRECTION('',(0.707106781186546,0.707106781186549,0.));
#2945=DIRECTION('',(0.,0.,-1.));
#2946=DIRECTION('',(0.707106781186546,0.707106781186549,0.));
#2947=DIRECTION('',(0.,0.,-1.));
#2948=DIRECTION('',(0.707106781186546,0.707106781186549,0.));
#2949=DIRECTION('',(0.,0.,-1.));
#2950=DIRECTION('center_axis',(0.,0.,1.));
#2951=DIRECTION('ref_axis',(-0.99412594534969,0.10822940812268,0.));
#2952=DIRECTION('center_axis',(0.,0.,1.));
#2953=DIRECTION('ref_axis',(-1.,0.,0.));
#2954=DIRECTION('',(0.,0.,1.));
#2955=DIRECTION('center_axis',(0.,0.,1.));
#2956=DIRECTION('ref_axis',(-1.,0.,0.));
#2957=DIRECTION('center_axis',(-0.707106781186546,-0.707106781186549,0.));
#2958=DIRECTION('ref_axis',(0.707106781186549,-0.707106781186546,0.));
#2959=DIRECTION('',(-0.707106781186549,0.707106781186546,0.));
#2960=DIRECTION('',(0.,0.,-1.));
#2961=DIRECTION('',(-0.707106781186549,0.707106781186546,0.));
#2962=DIRECTION('',(0.,0.,-1.));
#2963=DIRECTION('center_axis',(0.537299608346827,0.843391445812884,0.));
#2964=DIRECTION('ref_axis',(-0.843391445812884,0.537299608346827,0.));
#2965=DIRECTION('',(0.843391445812883,-0.537299608346827,0.));
#2966=DIRECTION('',(0.,0.,-1.));
#2967=DIRECTION('',(0.843391445812883,-0.537299608346827,0.));
#2968=DIRECTION('center_axis',(-0.707106781186552,0.707106781186543,0.));
#2969=DIRECTION('ref_axis',(-0.707106781186543,-0.707106781186552,0.));
#2970=DIRECTION('',(0.707106781186543,0.707106781186552,0.));
#2971=DIRECTION('',(0.,0.,-1.));
#2972=DIRECTION('',(0.707106781186543,0.707106781186552,0.));
#2973=DIRECTION('center_axis',(0.707106781186547,0.707106781186548,0.));
#2974=DIRECTION('ref_axis',(-0.707106781186548,0.707106781186547,0.));
#2975=DIRECTION('',(0.707106781186548,-0.707106781186547,0.));
#2976=DIRECTION('',(0.,0.,-1.));
#2977=DIRECTION('',(0.707106781186548,-0.707106781186547,0.));
#2978=DIRECTION('center_axis',(0.965925826289068,0.258819045102523,0.));
#2979=DIRECTION('ref_axis',(-0.258819045102523,0.965925826289068,0.));
#2980=DIRECTION('',(0.258819045102523,-0.965925826289068,0.));
#2981=DIRECTION('',(0.,0.,-1.));
#2982=DIRECTION('',(0.258819045102523,-0.965925826289068,0.));
#2983=DIRECTION('center_axis',(-0.707106781186541,0.707106781186554,0.));
#2984=DIRECTION('ref_axis',(-0.707106781186554,-0.707106781186541,0.));
#2985=DIRECTION('',(0.707106781186554,0.707106781186541,0.));
#2986=DIRECTION('',(0.,0.,-1.));
#2987=DIRECTION('',(0.707106781186554,0.707106781186541,0.));
#2988=DIRECTION('center_axis',(0.707106781186545,0.70710678118655,0.));
#2989=DIRECTION('ref_axis',(-0.70710678118655,0.707106781186545,0.));
#2990=DIRECTION('',(0.70710678118655,-0.707106781186545,0.));
#2991=DIRECTION('',(0.70710678118655,-0.707106781186545,0.));
#2992=DIRECTION('center_axis',(-0.707106781186546,-0.707106781186549,0.));
#2993=DIRECTION('ref_axis',(0.707106781186549,-0.707106781186546,0.));
#2994=DIRECTION('',(-0.707106781186549,0.707106781186546,0.));
#2995=DIRECTION('',(0.,0.,1.));
#2996=DIRECTION('',(-0.707106781186549,0.707106781186546,0.));
#2997=DIRECTION('center_axis',(0.,0.,-1.));
#2998=DIRECTION('ref_axis',(-1.,0.,0.));
#2999=DIRECTION('center_axis',(0.,0.,1.));
#3000=DIRECTION('ref_axis',(-1.,0.,0.));
#3001=DIRECTION('',(0.965925826289068,-0.258819045102521,0.));
#3002=DIRECTION('center_axis',(0.,0.,-1.));
#3003=DIRECTION('ref_axis',(-1.,0.,0.));
#3004=DIRECTION('',(0.965925826289068,-0.258819045102521,0.));
#3005=DIRECTION('center_axis',(0.258819045102521,0.965925826289068,0.));
#3006=DIRECTION('ref_axis',(-0.965925826289068,0.258819045102521,0.));
#3007=DIRECTION('',(0.965925826289068,-0.258819045102521,0.));
#3008=DIRECTION('',(0.,0.,1.));
#3009=DIRECTION('',(0.965925826289068,-0.258819045102521,0.));
#3010=DIRECTION('',(0.,0.,1.));
#3011=DIRECTION('center_axis',(0.,0.,1.));
#3012=DIRECTION('ref_axis',(-0.99412594534969,0.10822940812268,0.));
#3013=DIRECTION('center_axis',(0.,0.,1.));
#3014=DIRECTION('ref_axis',(-1.,0.,0.));
#3015=DIRECTION('center_axis',(0.707106781186548,-0.707106781186547,0.));
#3016=DIRECTION('ref_axis',(0.,0.,-1.));
#3017=DIRECTION('',(0.707106781186547,0.707106781186548,0.));
#3018=DIRECTION('',(0.,0.,-1.));
#3019=DIRECTION('',(0.707106781186547,0.707106781186548,0.));
#3020=DIRECTION('center_axis',(0.707106781186549,-0.707106781186546,0.));
#3021=DIRECTION('ref_axis',(0.,0.,-1.));
#3022=DIRECTION('',(0.707106781186546,0.707106781186549,0.));
#3023=DIRECTION('',(0.,0.,-1.));
#3024=DIRECTION('',(0.707106781186546,0.707106781186549,0.));
#3025=DIRECTION('center_axis',(-0.707106781186546,-0.707106781186549,0.));
#3026=DIRECTION('ref_axis',(0.707106781186549,-0.707106781186546,0.));
#3027=DIRECTION('',(-0.707106781186549,0.707106781186546,0.));
#3028=DIRECTION('',(-0.707106781186549,0.707106781186546,0.));
#3029=DIRECTION('center_axis',(-0.707106781186546,-0.707106781186549,0.));
#3030=DIRECTION('ref_axis',(0.707106781186549,-0.707106781186546,0.));
#3031=DIRECTION('',(-0.707106781186549,0.707106781186546,0.));
#3032=DIRECTION('',(-0.707106781186549,0.707106781186546,0.));
#3033=DIRECTION('center_axis',(0.,0.,-1.));
#3034=DIRECTION('ref_axis',(-1.,0.,0.));
#3035=DIRECTION('center_axis',(0.,0.,-1.));
#3036=DIRECTION('ref_axis',(-1.,0.,0.));
#3037=DIRECTION('center_axis',(0.,0.,1.));
#3038=DIRECTION('ref_axis',(1.,0.,0.));
#3039=DIRECTION('center_axis',(0.,0.,1.));
#3040=DIRECTION('ref_axis',(1.,0.,0.));
#3538=CARTESIAN_POINT('',(0.,0.,0.));
#3539=CARTESIAN_POINT('Origin',(0.,0.,-4.5));
#3540=CARTESIAN_POINT('',(-1.25,-1.53080849893419E-16,4.));
#3541=CARTESIAN_POINT('Origin',(0.,0.,4.));
#3542=CARTESIAN_POINT('',(-1.25,-1.53080849893419E-16,4.5));
#3543=CARTESIAN_POINT('',(-1.25,-1.53080849893419E-16,-4.5));
#3544=CARTESIAN_POINT('Origin',(0.,0.,4.5));
#3545=CARTESIAN_POINT('Origin',(0.,0.,-4.5));
#3546=CARTESIAN_POINT('',(-1.25,-1.53080849893419E-16,-4.5));
#3547=CARTESIAN_POINT('Origin',(0.,0.,-4.5));
#3548=CARTESIAN_POINT('',(-1.25,-1.53080849893419E-16,-4.));
#3549=CARTESIAN_POINT('',(-1.25,-1.53080849893419E-16,-4.5));
#3550=CARTESIAN_POINT('Origin',(0.,0.,-4.));
#3551=CARTESIAN_POINT('Origin',(0.,0.,5.));
#3552=CARTESIAN_POINT('',(5.3033008588991,5.30330085889912,5.));
#3553=CARTESIAN_POINT('',(-4.02974706260121,-6.32543584359663,5.));
#3554=CARTESIAN_POINT('Origin',(0.,0.,5.));
#3555=CARTESIAN_POINT('',(5.3033008588991,5.30330085889912,4.));
#3556=CARTESIAN_POINT('',(5.3033008588991,5.30330085889912,5.));
#3557=CARTESIAN_POINT('',(-4.02974706260121,-6.32543584359663,4.));
#3558=CARTESIAN_POINT('Origin',(0.,0.,4.));
#3559=CARTESIAN_POINT('',(-4.02974706260121,-6.32543584359663,5.));
#3560=CARTESIAN_POINT('Origin',(7.7979471106944,2.10154782591728,-85.1116718670025));
#3561=CARTESIAN_POINT('',(7.82039743172835,1.60205209712125,4.));
#3562=CARTESIAN_POINT('',(8.15150050128767,2.45510121651055,4.));
#3563=CARTESIAN_POINT('Origin',(7.7979471106944,2.10154782591728,4.));
#3564=CARTESIAN_POINT('',(8.15150050128767,2.45510121651055,5.));
#3565=CARTESIAN_POINT('',(8.15150050128767,2.45510121651055,-5.));
#3566=CARTESIAN_POINT('',(7.82039743172835,1.60205209712125,5.));
#3567=CARTESIAN_POINT('Origin',(7.7979471106944,2.10154782591728,5.));
#3568=CARTESIAN_POINT('',(7.82039743172835,1.60205209712125,-85.1116718670025));
#3569=CARTESIAN_POINT('Origin',(7.7979471106944,2.10154782591728,-85.1116718670025));
#3570=CARTESIAN_POINT('',(8.15150050128767,2.45510121651055,-5.));
#3571=CARTESIAN_POINT('',(7.82039743172835,1.60205209712125,-5.));
#3572=CARTESIAN_POINT('Origin',(7.7979471106944,2.10154782591728,-5.));
#3573=CARTESIAN_POINT('',(8.15150050128767,2.45510121651055,-4.));
#3574=CARTESIAN_POINT('',(8.15150050128767,2.45510121651055,-5.));
#3575=CARTESIAN_POINT('',(7.82039743172835,1.60205209712125,-4.));
#3576=CARTESIAN_POINT('Origin',(7.7979471106944,2.10154782591728,-4.));
#3577=CARTESIAN_POINT('',(7.82039743172835,1.60205209712125,-85.1116718670025));
#3578=CARTESIAN_POINT('Origin',(0.,0.,5.));
#3579=CARTESIAN_POINT('',(5.3033008588991,5.30330085889912,-4.));
#3580=CARTESIAN_POINT('',(-4.02974706260121,-6.32543584359663,-4.));
#3581=CARTESIAN_POINT('Origin',(0.,0.,-4.));
#3582=CARTESIAN_POINT('',(5.3033008588991,5.30330085889912,-5.));
#3583=CARTESIAN_POINT('',(5.3033008588991,5.30330085889912,5.));
#3584=CARTESIAN_POINT('',(-4.02974706260121,-6.32543584359663,-5.));
#3585=CARTESIAN_POINT('Origin',(0.,0.,-5.));
#3586=CARTESIAN_POINT('',(-4.02974706260121,-6.32543584359663,5.));
#3587=CARTESIAN_POINT('Origin',(17.3220165268891,-19.9280094422533,5.));
#3588=CARTESIAN_POINT('',(17.3220165268891,-19.9280094422533,-4.));
#3589=CARTESIAN_POINT('',(-4.02974706260121,-6.32543584359663,-4.));
#3590=CARTESIAN_POINT('',(17.3220165268891,-19.9280094422533,-5.));
#3591=CARTESIAN_POINT('',(17.3220165268891,-19.9280094422533,-5.));
#3592=CARTESIAN_POINT('',(17.3220165268891,-19.9280094422533,5.));
#3593=CARTESIAN_POINT('Origin',(20.3927799375376,-16.8572460316048,5.));
#3594=CARTESIAN_POINT('',(20.3927799375376,-16.8572460316048,-4.));
#3595=CARTESIAN_POINT('',(18.6250129845713,-18.6250129845711,-4.));
#3596=CARTESIAN_POINT('',(20.3927799375376,-16.8572460316048,-5.));
#3597=CARTESIAN_POINT('',(20.3927799375376,-16.8572460316048,-5.));
#3598=CARTESIAN_POINT('',(20.3927799375376,-16.8572460316048,5.));
#3599=CARTESIAN_POINT('Origin',(23.9283138434703,-20.3927799375375,5.));
#3600=CARTESIAN_POINT('',(23.9283138434703,-20.3927799375375,-4.));
#3601=CARTESIAN_POINT('',(1.76776695296638,1.76776695296638,-4.));
#3602=CARTESIAN_POINT('',(23.9283138434703,-20.3927799375375,-5.));
#3603=CARTESIAN_POINT('',(23.9283138434703,-20.3927799375375,-5.));
#3604=CARTESIAN_POINT('',(23.9283138434703,-20.3927799375375,5.));
#3605=CARTESIAN_POINT('Origin',(26.5165042944955,-30.0520382004282,5.));
#3606=CARTESIAN_POINT('',(26.5165042944955,-30.0520382004282,-4.));
#3607=CARTESIAN_POINT('',(17.2272257664368,4.61602123194541,-4.));
#3608=CARTESIAN_POINT('',(26.5165042944955,-30.0520382004282,-5.));
#3609=CARTESIAN_POINT('',(26.5165042944955,-30.0520382004282,-5.));
#3610=CARTESIAN_POINT('',(26.5165042944955,-30.0520382004282,5.));
#3611=CARTESIAN_POINT('Origin',(30.0520382004283,-26.5165042944955,5.));
#3612=CARTESIAN_POINT('',(30.0520382004283,-26.5165042944955,-4.));
#3613=CARTESIAN_POINT('',(28.2842712474616,-28.2842712474621,-4.));
#3614=CARTESIAN_POINT('',(30.0520382004283,-26.5165042944955,-5.));
#3615=CARTESIAN_POINT('',(30.0520382004283,-26.5165042944955,-5.));
#3616=CARTESIAN_POINT('',(30.0520382004283,-26.5165042944955,5.));
#3617=CARTESIAN_POINT('Origin',(37.1231060122938,-33.5875721063609,5.));
#3618=CARTESIAN_POINT('',(37.1231060122938,-33.5875721063609,-4.));
#3619=CARTESIAN_POINT('',(1.76776695296631,1.76776695296632,-4.));
#3620=CARTESIAN_POINT('',(37.1231060122938,-33.5875721063609,-5.));
#3621=CARTESIAN_POINT('',(37.1231060122938,-33.5875721063609,-5.));
#3622=CARTESIAN_POINT('',(37.1231060122938,-33.5875721063609,5.));
#3623=CARTESIAN_POINT('Origin',(40.6586399182266,-30.0520382004282,5.));
#3624=CARTESIAN_POINT('',(39.95153313704,-30.7591449816147,-4.));
#3625=CARTESIAN_POINT('',(35.3553390593274,-35.3553390593273,-4.));
#3626=CARTESIAN_POINT('',(40.6586399182266,-30.0520382004282,-5.));
#3627=CARTESIAN_POINT('',(40.6586399182266,-30.0520382004282,-5.));
#3628=CARTESIAN_POINT('',(40.6586399182266,-30.0520382004282,5.));
#3629=CARTESIAN_POINT('',(40.6586399182266,-30.0520382004282,5.));
#3630=CARTESIAN_POINT('',(37.1231060122938,-33.5875721063609,5.));
#3631=CARTESIAN_POINT('',(40.6586399182266,-30.0520382004282,5.));
#3632=CARTESIAN_POINT('',(37.1231060122938,-33.5875721063609,4.));
#3633=CARTESIAN_POINT('',(37.1231060122938,-33.5875721063609,5.));
#3634=CARTESIAN_POINT('',(39.95153313704,-30.7591449816147,4.));
#3635=CARTESIAN_POINT('',(35.3553390593274,-35.3553390593273,4.));
#3636=CARTESIAN_POINT('',(39.95153313704,-30.7591449816147,5.));
#3637=CARTESIAN_POINT('Origin',(8.,-2.39391373324695,-85.1116718670025));
#3638=CARTESIAN_POINT('',(6.96472381958992,-6.25761703840322,-4.));
#3639=CARTESIAN_POINT('Origin',(8.,-2.39391373324695,-4.));
#3640=CARTESIAN_POINT('',(6.96472381958992,-6.25761703840322,-5.));
#3641=CARTESIAN_POINT('',(6.96472381958992,-6.25761703840322,-85.1116718670025));
#3642=CARTESIAN_POINT('Origin',(8.,-2.39391373324695,-5.));
#3643=CARTESIAN_POINT('Origin',(5.3033008588991,5.30330085889912,5.));
#3644=CARTESIAN_POINT('',(5.3033008588991,5.30330085889912,5.));
#3645=CARTESIAN_POINT('',(8.15150050128767,2.45510121651055,-5.));
#3646=CARTESIAN_POINT('',(5.3033008588991,5.30330085889912,-5.));
#3647=CARTESIAN_POINT('',(5.3033008588991,5.30330085889912,5.));
#3648=CARTESIAN_POINT('Origin',(17.3220165268891,-19.9280094422533,5.));
#3649=CARTESIAN_POINT('',(17.3220165268891,-19.9280094422533,4.));
#3650=CARTESIAN_POINT('',(-4.02974706260121,-6.32543584359663,4.));
#3651=CARTESIAN_POINT('',(17.3220165268891,-19.9280094422533,5.));
#3652=CARTESIAN_POINT('',(17.3220165268891,-19.9280094422533,5.));
#3653=CARTESIAN_POINT('',(17.3220165268891,-19.9280094422533,5.));
#3654=CARTESIAN_POINT('Origin',(20.3927799375376,-16.8572460316048,5.));
#3655=CARTESIAN_POINT('',(20.3927799375376,-16.8572460316048,4.));
#3656=CARTESIAN_POINT('',(18.6250129845713,-18.6250129845711,4.));
#3657=CARTESIAN_POINT('',(20.3927799375376,-16.8572460316048,5.));
#3658=CARTESIAN_POINT('',(20.3927799375376,-16.8572460316048,5.));
#3659=CARTESIAN_POINT('',(20.3927799375376,-16.8572460316048,5.));
#3660=CARTESIAN_POINT('Origin',(23.9283138434703,-20.3927799375375,5.));
#3661=CARTESIAN_POINT('',(23.9283138434703,-20.3927799375375,4.));
#3662=CARTESIAN_POINT('',(1.76776695296638,1.76776695296638,4.));
#3663=CARTESIAN_POINT('',(23.9283138434703,-20.3927799375375,5.));
#3664=CARTESIAN_POINT('',(23.9283138434703,-20.3927799375375,5.));
#3665=CARTESIAN_POINT('',(23.9283138434703,-20.3927799375375,5.));
#3666=CARTESIAN_POINT('Origin',(26.5165042944955,-30.0520382004282,5.));
#3667=CARTESIAN_POINT('',(26.5165042944955,-30.0520382004282,4.));
#3668=CARTESIAN_POINT('',(17.2272257664368,4.61602123194541,4.));
#3669=CARTESIAN_POINT('',(26.5165042944955,-30.0520382004282,5.));
#3670=CARTESIAN_POINT('',(26.5165042944955,-30.0520382004282,5.));
#3671=CARTESIAN_POINT('',(26.5165042944955,-30.0520382004282,5.));
#3672=CARTESIAN_POINT('Origin',(30.0520382004283,-26.5165042944955,5.));
#3673=CARTESIAN_POINT('',(30.0520382004283,-26.5165042944955,4.));
#3674=CARTESIAN_POINT('',(28.2842712474616,-28.2842712474621,4.));
#3675=CARTESIAN_POINT('',(30.0520382004283,-26.5165042944955,5.));
#3676=CARTESIAN_POINT('',(30.0520382004283,-26.5165042944955,5.));
#3677=CARTESIAN_POINT('',(30.0520382004283,-26.5165042944955,5.));
#3678=CARTESIAN_POINT('Origin',(37.1231060122938,-33.5875721063609,5.));
#3679=CARTESIAN_POINT('',(1.76776695296631,1.76776695296632,4.));
#3680=CARTESIAN_POINT('',(37.1231060122938,-33.5875721063609,5.));
#3681=CARTESIAN_POINT('Origin',(5.3033008588991,5.30330085889912,5.));
#3682=CARTESIAN_POINT('',(20.4876853876369,-9.88108366983852,-5.));
#3683=CARTESIAN_POINT('',(5.3033008588991,5.30330085889912,-5.));
#3684=CARTESIAN_POINT('',(20.4876853876369,-9.88108366983852,5.));
#3685=CARTESIAN_POINT('',(20.4876853876369,-9.88108366983852,-85.1116718670025));
#3686=CARTESIAN_POINT('',(5.3033008588991,5.30330085889912,5.));
#3687=CARTESIAN_POINT('Origin',(0.,0.,5.));
#3688=CARTESIAN_POINT('',(6.96472381958992,-6.25761703840322,5.));
#3689=CARTESIAN_POINT('Origin',(8.,-2.39391373324695,5.));
#3690=CARTESIAN_POINT('',(-1.09785622885958,-4.09725522550989,5.));
#3691=CARTESIAN_POINT('Origin',(0.,0.,-5.));
#3692=CARTESIAN_POINT('',(-1.09785622885958,-4.09725522550989,-5.));
#3693=CARTESIAN_POINT('Origin',(20.4876853876369,-9.88108366983852,-85.1116718670025));
#3694=CARTESIAN_POINT('',(6.96472381958992,-6.25761703840322,4.));
#3695=CARTESIAN_POINT('',(18.5558337350586,-9.36344557963344,4.));
#3696=CARTESIAN_POINT('',(-1.09785622885958,-4.09725522550989,4.));
#3697=CARTESIAN_POINT('',(6.96472381958992,-6.25761703840322,-85.1116718670025));
#3698=CARTESIAN_POINT('',(18.5558337350586,-9.36344557963344,-4.));
#3699=CARTESIAN_POINT('',(-1.09785622885958,-4.09725522550989,-4.));
#3700=CARTESIAN_POINT('',(18.5558337350586,-9.36344557963344,-85.1116718670025));
#3701=CARTESIAN_POINT('Origin',(8.,-2.39391373324695,-85.1116718670025));
#3702=CARTESIAN_POINT('Origin',(8.,-2.39391373324695,4.));
#3703=CARTESIAN_POINT('Origin',(8.15150050128767,2.45510121651055,0.));
#3704=CARTESIAN_POINT('',(7.44439372010113,1.747994435324,4.));
#3705=CARTESIAN_POINT('',(8.15150050128767,2.45510121651055,4.));
#3706=CARTESIAN_POINT('',(7.44439372010113,1.747994435324,-4.));
#3707=CARTESIAN_POINT('',(7.44439372010113,1.747994435324,5.));
#3708=CARTESIAN_POINT('',(2.84819964238857,-2.84819964238856,-4.));
#3709=CARTESIAN_POINT('Origin',(5.3033008588991,5.30330085889912,0.));
#3710=CARTESIAN_POINT('',(4.59619407771255,4.59619407771257,-4.));
#3711=CARTESIAN_POINT('',(5.3033008588991,5.30330085889912,-4.));
#3712=CARTESIAN_POINT('',(4.59619407771255,4.59619407771257,4.));
#3713=CARTESIAN_POINT('',(4.59619407771255,4.59619407771257,0.));
#3714=CARTESIAN_POINT('',(5.3033008588991,5.30330085889912,4.));
#3715=CARTESIAN_POINT('Origin',(4.59619407771255,4.59619407771257,5.));
#3716=CARTESIAN_POINT('',(4.59619407771255,4.59619407771257,4.));
#3717=CARTESIAN_POINT('',(4.59619407771255,4.59619407771257,-4.));
#3718=CARTESIAN_POINT('Origin',(4.59619407771255,4.59619407771257,5.));
#3719=CARTESIAN_POINT('',(4.59619407771255,4.59619407771257,-4.));
#3720=CARTESIAN_POINT('',(4.59619407771255,4.59619407771257,4.));
#3721=CARTESIAN_POINT('Origin',(0.,0.,4.));
#3722=CARTESIAN_POINT('Origin',(0.,0.,-4.));
#3723=CARTESIAN_POINT('Origin',(0.,0.,-4.5));
#3724=CARTESIAN_POINT('Origin',(0.,0.,4.5));
#9548=UNCERTAINTY_MEASURE_WITH_UNIT(LENGTH_MEASURE(0.01),#9562,
'DISTANCE_ACCURACY_VALUE',
'Maximum model space distance between geometric entities at asserted c
onnectivities');
#9553=UNCERTAINTY_MEASURE_WITH_UNIT(LENGTH_MEASURE(0.01),#9562,
'DISTANCE_ACCURACY_VALUE',
'Maximum model space distance between geometric entities at asserted c
onnectivities');
#9556=(
GEOMETRIC_REPRESENTATION_CONTEXT(3)
GLOBAL_UNCERTAINTY_ASSIGNED_CONTEXT((#9548))
GLOBAL_UNIT_ASSIGNED_CONTEXT((#9562,#9564,#9565))
REPRESENTATION_CONTEXT('','3D')
);
#9561=(
GEOMETRIC_REPRESENTATION_CONTEXT(3)
GLOBAL_UNCERTAINTY_ASSIGNED_CONTEXT((#9553))
GLOBAL_UNIT_ASSIGNED_CONTEXT((#9562,#9564,#9565))
REPRESENTATION_CONTEXT('','3D')
);
#9562=(
LENGTH_UNIT()
NAMED_UNIT(*)
SI_UNIT(.MILLI.,.METRE.)
);
#9564=(
NAMED_UNIT(*)
PLANE_ANGLE_UNIT()
SI_UNIT($,.RADIAN.)
);
#9565=(
NAMED_UNIT(*)
SI_UNIT($,.STERADIAN.)
SOLID_ANGLE_UNIT()
);
#9568=SHAPE_DEFINITION_REPRESENTATION(#9575,#9588);
#9575=PRODUCT_DEFINITION_SHAPE('',$,#9596);
#9588=SHAPE_REPRESENTATION('',(#2539),#9556);
#9593=PRODUCT_DEFINITION_CONTEXT('part definition',#9616,'design');
#9596=PRODUCT_DEFINITION('fulcrum','fulcrum',#9603,#9593);
#9603=PRODUCT_DEFINITION_FORMATION('',$,#9620);
#9616=APPLICATION_CONTEXT(
'Core Data for Automotive Mechanical Design Process');
#9617=PRODUCT_CONTEXT('part definition',#9616,'mechanical');
#9620=PRODUCT('fulcrum','fulcrum',$,(#9617));
#9627=PRESENTATION_STYLE_ASSIGNMENT((#9632));
#9632=SURFACE_STYLE_USAGE(.BOTH.,#9637);
#9637=SURFACE_SIDE_STYLE('',(#9642));
#9642=SURFACE_STYLE_FILL_AREA(#9647);
#9647=FILL_AREA_STYLE('Opaque(97,158,199)',(#9652));
#9652=FILL_AREA_STYLE_COLOUR('Opaque(97,158,199)',#9657);
#9657=COLOUR_RGB('Opaque(97,158,199)',0.380392156862745,0.619607843137255,
0.780392156862745);
ENDSEC;
END-ISO-10303-21;
